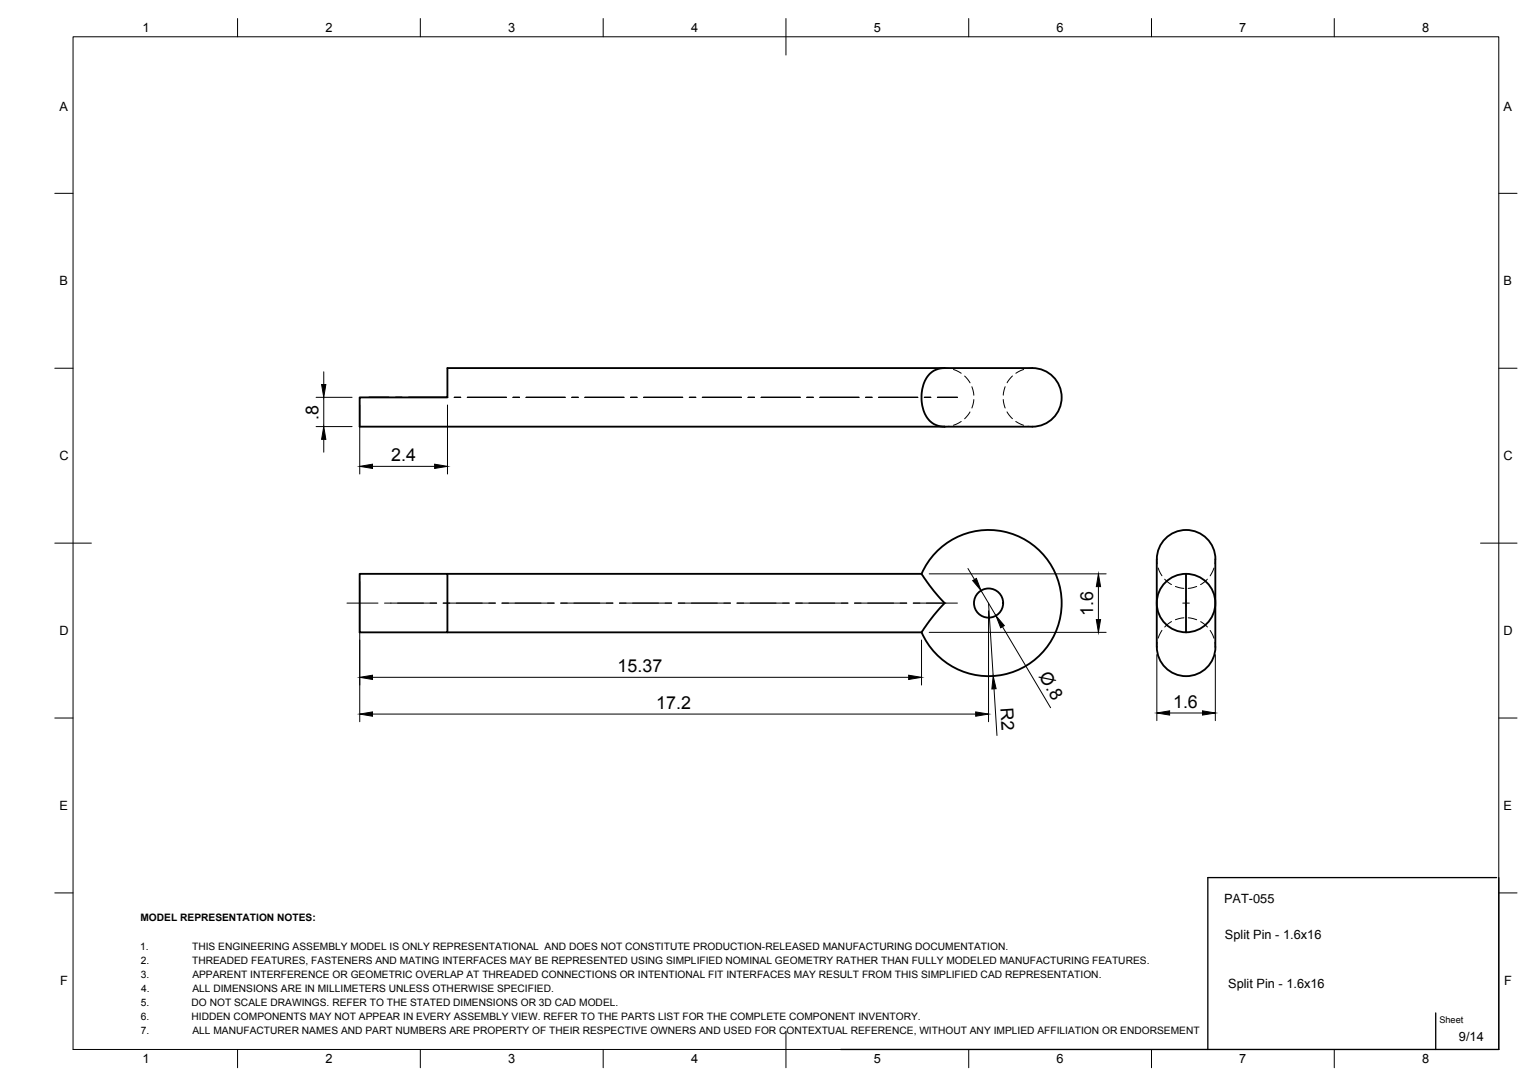
ISO-10303-21;
HEADER;
/* Generated by software containing ST-Developer
 * from STEP Tools, Inc. (www.steptools.com) 
 */

FILE_DESCRIPTION(
/* description */ ('Hinged panel with latch'),
/* implementation_level */ '2;1');

FILE_NAME(
/* name */ 'Split Pin - 1.6x16.step',
/* time_stamp */ '2026-10-27T20:36:01-07:00',
/* author */ (''),
/* organization */ (''),
/* preprocessor_version */ 'ST-DEVELOPER v20.2',
/* originating_system */ 'Autodesk Translation Framework v15.17.0.0',
/* authorisation */ '');

FILE_SCHEMA (('AUTOMOTIVE_DESIGN { 1 0 10303 214 3 1 1 }'));
ENDSEC;

DATA;
#10=MECHANICAL_DESIGN_GEOMETRIC_PRESENTATION_REPRESENTATION('',(#301),#6743);
#239=TOROIDAL_SURFACE('',#4113,0.12,0.08);
#262=B_SPLINE_CURVE_WITH_KNOTS('',3,(#5988,#5989,#5990,#5991,#5992,#5993,
#5994,#5995,#5996,#5997,#5998,#5999,#6000,#6001,#6002,#6003,#6004,#6005,
#6006,#6007,#6008,#6009,#6010,#6011,#6012,#6013),.UNSPECIFIED.,.F.,.F.,
(4,2,2,2,2,2,2,2,2,2,2,2,4),(-0.00054581412719389,0.,0.0281583564005144,
0.0618496465371181,0.0905865724114538,0.120694112793616,0.144966158459363,
0.16923820412511,0.199345744507272,0.228082670381608,0.261773960518212,
0.289932316918681,0.290478131045882),.UNSPECIFIED.);
#263=B_SPLINE_CURVE_WITH_KNOTS('',3,(#6014,#6015,#6016,#6017,#6018,#6019,
#6020,#6021,#6022,#6023,#6024,#6025,#6026,#6027,#6028,#6029,#6030,#6031,
#6032,#6033,#6034,#6035,#6036,#6037,#6038,#6039),.UNSPECIFIED.,.F.,.F.,
(4,2,2,2,2,2,2,2,2,2,2,2,4),(-0.000545814127196571,0.,0.0281583564006391,
0.0618496465374156,0.0905865724118984,0.120694112794215,0.144966158460086,
0.169238204125958,0.199345744508275,0.228082670382758,0.261773960519534,
0.289932316920171,0.29047813104737),.UNSPECIFIED.);
#269=SHAPE_REPRESENTATION_RELATIONSHIP('SRR','None',#6844,#285);
#285=ADVANCED_BREP_SHAPE_REPRESENTATION('',(#317),#6730);
#301=STYLED_ITEM('',(#7003),#317);
#317=MANIFOLD_SOLID_BREP('Body1',#3803);
#343=FACE_BOUND('',#831,.T.);
#439=PLANE('',#4116);
#440=PLANE('',#4118);
#441=PLANE('',#4122);
#606=FACE_OUTER_BOUND('',#830,.T.);
#607=FACE_OUTER_BOUND('',#832,.T.);
#608=FACE_OUTER_BOUND('',#833,.T.);
#609=FACE_OUTER_BOUND('',#834,.T.);
#610=FACE_OUTER_BOUND('',#835,.T.);
#830=EDGE_LOOP('',(#3024,#3025,#3026,#3027));
#831=EDGE_LOOP('',(#3028,#3029));
#832=EDGE_LOOP('',(#3030,#3031));
#833=EDGE_LOOP('',(#3032,#3033,#3034,#3035));
#834=EDGE_LOOP('',(#3036,#3037,#3038,#3039,#3040,#3041,#3042,#3043,#3044));
#835=EDGE_LOOP('',(#3045,#3046,#3047));
#1167=LINE('',#6044,#1525);
#1168=LINE('',#6047,#1526);
#1169=LINE('',#6049,#1527);
#1170=LINE('',#6050,#1528);
#1171=LINE('',#6054,#1529);
#1525=VECTOR('',#4797,1.);
#1526=VECTOR('',#4800,1.);
#1527=VECTOR('',#4801,1.);
#1528=VECTOR('',#4802,1.);
#1529=VECTOR('',#4807,0.08);
#1726=CIRCLE('',#4114,0.08);
#1727=CIRCLE('',#4115,0.04);
#1728=CIRCLE('',#4117,0.08);
#1729=CIRCLE('',#4120,0.08);
#1730=CIRCLE('',#4121,0.08);
#1935=VERTEX_POINT('',#5983);
#1936=VERTEX_POINT('',#5986);
#1937=VERTEX_POINT('',#5987);
#1938=VERTEX_POINT('',#6041);
#1939=VERTEX_POINT('',#6042);
#1940=VERTEX_POINT('',#6046);
#1941=VERTEX_POINT('',#6048);
#1942=VERTEX_POINT('',#6052);
#2324=EDGE_CURVE('',#1935,#1935,#1726,.T.);
#2325=EDGE_CURVE('',#1935,#1935,#1727,.T.);
#2326=EDGE_CURVE('',#1936,#1937,#262,.T.);
#2327=EDGE_CURVE('',#1937,#1936,#263,.T.);
#2328=EDGE_CURVE('',#1938,#1939,#1728,.T.);
#2329=EDGE_CURVE('',#1938,#1939,#1167,.T.);
#2330=EDGE_CURVE('',#1939,#1940,#1168,.T.);
#2331=EDGE_CURVE('',#1941,#1940,#1169,.T.);
#2332=EDGE_CURVE('',#1938,#1941,#1170,.T.);
#2333=EDGE_CURVE('',#1942,#1941,#1729,.T.);
#2334=EDGE_CURVE('',#1942,#1937,#1171,.T.);
#2335=EDGE_CURVE('',#1940,#1942,#1730,.T.);
#3024=ORIENTED_EDGE('',*,*,#2324,.F.);
#3025=ORIENTED_EDGE('',*,*,#2325,.T.);
#3026=ORIENTED_EDGE('',*,*,#2324,.T.);
#3027=ORIENTED_EDGE('',*,*,#2325,.F.);
#3028=ORIENTED_EDGE('',*,*,#2326,.F.);
#3029=ORIENTED_EDGE('',*,*,#2327,.F.);
#3030=ORIENTED_EDGE('',*,*,#2328,.T.);
#3031=ORIENTED_EDGE('',*,*,#2329,.F.);
#3032=ORIENTED_EDGE('',*,*,#2329,.T.);
#3033=ORIENTED_EDGE('',*,*,#2330,.T.);
#3034=ORIENTED_EDGE('',*,*,#2331,.F.);
#3035=ORIENTED_EDGE('',*,*,#2332,.F.);
#3036=ORIENTED_EDGE('',*,*,#2328,.F.);
#3037=ORIENTED_EDGE('',*,*,#2332,.T.);
#3038=ORIENTED_EDGE('',*,*,#2333,.F.);
#3039=ORIENTED_EDGE('',*,*,#2334,.T.);
#3040=ORIENTED_EDGE('',*,*,#2327,.T.);
#3041=ORIENTED_EDGE('',*,*,#2326,.T.);
#3042=ORIENTED_EDGE('',*,*,#2334,.F.);
#3043=ORIENTED_EDGE('',*,*,#2335,.F.);
#3044=ORIENTED_EDGE('',*,*,#2330,.F.);
#3045=ORIENTED_EDGE('',*,*,#2335,.T.);
#3046=ORIENTED_EDGE('',*,*,#2333,.T.);
#3047=ORIENTED_EDGE('',*,*,#2331,.T.);
#3570=CYLINDRICAL_SURFACE('',#4119,0.08);
#3675=ADVANCED_FACE('',(#606,#343),#239,.T.);
#3676=ADVANCED_FACE('',(#607),#439,.F.);
#3677=ADVANCED_FACE('',(#608),#440,.T.);
#3678=ADVANCED_FACE('',(#609),#3570,.T.);
#3679=ADVANCED_FACE('',(#610),#441,.F.);
#3803=CLOSED_SHELL('',(#3675,#3676,#3677,#3678,#3679));
#4112=AXIS2_PLACEMENT_3D('',#5981,#4785,#4786);
#4113=AXIS2_PLACEMENT_3D('',#5982,#4787,#4788);
#4114=AXIS2_PLACEMENT_3D('',#5984,#4789,#4790);
#4115=AXIS2_PLACEMENT_3D('',#5985,#4791,#4792);
#4116=AXIS2_PLACEMENT_3D('',#6040,#4793,#4794);
#4117=AXIS2_PLACEMENT_3D('',#6043,#4795,#4796);
#4118=AXIS2_PLACEMENT_3D('',#6045,#4798,#4799);
#4119=AXIS2_PLACEMENT_3D('',#6051,#4803,#4804);
#4120=AXIS2_PLACEMENT_3D('',#6053,#4805,#4806);
#4121=AXIS2_PLACEMENT_3D('',#6055,#4808,#4809);
#4122=AXIS2_PLACEMENT_3D('',#6056,#4810,#4811);
#4785=DIRECTION('axis',(0.,0.,1.));
#4786=DIRECTION('refdir',(1.,0.,0.));
#4787=DIRECTION('center_axis',(-1.,0.,0.));
#4788=DIRECTION('ref_axis',(0.,0.,1.));
#4789=DIRECTION('center_axis',(0.,-1.,1.38777878078145E-16));
#4790=DIRECTION('ref_axis',(0.,-1.38777878078145E-16,-1.));
#4791=DIRECTION('center_axis',(1.,0.,0.));
#4792=DIRECTION('ref_axis',(0.,0.,1.));
#4793=DIRECTION('center_axis',(0.,1.,0.));
#4794=DIRECTION('ref_axis',(1.,0.,0.));
#4795=DIRECTION('center_axis',(0.,-1.,0.));
#4796=DIRECTION('ref_axis',(1.,0.,0.));
#4797=DIRECTION('',(0.,0.,1.));
#4798=DIRECTION('center_axis',(1.,0.,0.));
#4799=DIRECTION('ref_axis',(0.,0.,1.));
#4800=DIRECTION('',(0.,-1.,0.));
#4801=DIRECTION('',(0.,0.,1.));
#4802=DIRECTION('',(0.,-1.,0.));
#4803=DIRECTION('center_axis',(0.,-1.,0.));
#4804=DIRECTION('ref_axis',(1.,0.,0.));
#4805=DIRECTION('center_axis',(0.,-1.,0.));
#4806=DIRECTION('ref_axis',(1.,0.,0.));
#4807=DIRECTION('',(0.,1.,0.));
#4808=DIRECTION('center_axis',(0.,-1.,0.));
#4809=DIRECTION('ref_axis',(1.,0.,0.));
#4810=DIRECTION('center_axis',(0.,1.,0.));
#4811=DIRECTION('ref_axis',(1.,0.,0.));
#5981=CARTESIAN_POINT('',(0.,0.,0.));
#5982=CARTESIAN_POINT('Origin',(0.,0.12,0.));
#5983=CARTESIAN_POINT('',(-9.79717439317883E-18,0.12,-0.04));
#5984=CARTESIAN_POINT('Origin',(0.,0.12,-0.12));
#5985=CARTESIAN_POINT('Origin',(9.79717439317883E-18,0.12,0.));
#5986=CARTESIAN_POINT('',(0.08,-4.89858719658941E-18,7.34788079488412E-18));
#5987=CARTESIAN_POINT('',(-0.08,-4.89858719658941E-18,7.34788079488412E-18));
#5988=CARTESIAN_POINT('Ctrl Pts',(0.08,-4.89858719658941E-18,7.34788079488412E-18));
#5989=CARTESIAN_POINT('Ctrl Pts',(0.08,-0.00012864962353541,0.000128649623535413));
#5990=CARTESIAN_POINT('Ctrl Pts',(0.0799996896739287,-0.00025719571182076,
0.000257402596003253));
#5991=CARTESIAN_POINT('Ctrl Pts',(0.0799669711262291,-0.00701193164572964,
0.00703384588894362));
#5992=CARTESIAN_POINT('Ctrl Pts',(0.0791054994909294,-0.0133457972655825,
0.0139383126556792));
#5993=CARTESIAN_POINT('Ctrl Pts',(0.0749700088488058,-0.0265076530862524,
0.0292212026164895));
#5994=CARTESIAN_POINT('Ctrl Pts',(0.0712702072865517,-0.0331317062461458,
0.0375603420117568));
#5995=CARTESIAN_POINT('Ctrl Pts',(0.0612858949407667,-0.0440683985740427,
0.0520545604187517));
#5996=CARTESIAN_POINT('Ctrl Pts',(0.0555090276731744,-0.0485199197794574,
0.0582717815295611));
#5997=CARTESIAN_POINT('Ctrl Pts',(0.0412398082144208,-0.0561090538733877,
0.0691638397919718));
#5998=CARTESIAN_POINT('Ctrl Pts',(0.0327878980890048,-0.059089642483296,
0.0736229049587921));
#5999=CARTESIAN_POINT('Ctrl Pts',(0.0159233027310102,-0.0625179833270725,
0.0787936360751706));
#6000=CARTESIAN_POINT('Ctrl Pts',(0.00801661414593076,-0.0633030277982336,
0.08));
#6001=CARTESIAN_POINT('Ctrl Pts',(-0.00801661414593074,-0.0633030277982336,
0.08));
#6002=CARTESIAN_POINT('Ctrl Pts',(-0.0159233027310102,-0.0625179833270726,
0.0787936360751706));
#6003=CARTESIAN_POINT('Ctrl Pts',(-0.0327878980890049,-0.059089642483296,
0.0736229049587921));
#6004=CARTESIAN_POINT('Ctrl Pts',(-0.0412398082144209,-0.0561090538733877,
0.0691638397919717));
#6005=CARTESIAN_POINT('Ctrl Pts',(-0.0555090276731744,-0.0485199197794574,
0.0582717815295611));
#6006=CARTESIAN_POINT('Ctrl Pts',(-0.0612858949407667,-0.0440683985740427,
0.0520545604187517));
#6007=CARTESIAN_POINT('Ctrl Pts',(-0.0712702072865517,-0.0331317062461458,
0.0375603420117568));
#6008=CARTESIAN_POINT('Ctrl Pts',(-0.0749700088488058,-0.0265076530862524,
0.0292212026164895));
#6009=CARTESIAN_POINT('Ctrl Pts',(-0.0791054994909264,-0.0133457972655921,
0.0139383126556903));
#6010=CARTESIAN_POINT('Ctrl Pts',(-0.0799669711262287,-0.00701193164579759,
0.0070338458890125));
#6011=CARTESIAN_POINT('Ctrl Pts',(-0.0799996896739287,-0.000257195711817665,
0.000257402596000083));
#6012=CARTESIAN_POINT('Ctrl Pts',(-0.08,-0.000128649623538514,0.000128649623538516));
#6013=CARTESIAN_POINT('Ctrl Pts',(-0.08,-4.89858719658941E-18,7.34788079488412E-18));
#6014=CARTESIAN_POINT('Ctrl Pts',(-0.08,-4.89858719658941E-18,7.34788079488412E-18));
#6015=CARTESIAN_POINT('Ctrl Pts',(-0.08,-0.000128649623536042,-0.00012864962353603));
#6016=CARTESIAN_POINT('Ctrl Pts',(-0.0799996896739287,-0.000257195711820127,
-0.000257402596002604));
#6017=CARTESIAN_POINT('Ctrl Pts',(-0.0799669711262289,-0.0070119316457589,
-0.00703384588897312));
#6018=CARTESIAN_POINT('Ctrl Pts',(-0.0791054994909281,-0.0133457972655867,
-0.0139383126556841));
#6019=CARTESIAN_POINT('Ctrl Pts',(-0.0749700088488058,-0.0265076530862525,
-0.0292212026164896));
#6020=CARTESIAN_POINT('Ctrl Pts',(-0.0712702072865516,-0.0331317062461459,
-0.0375603420117568));
#6021=CARTESIAN_POINT('Ctrl Pts',(-0.0612858949407667,-0.0440683985740427,
-0.0520545604187517));
#6022=CARTESIAN_POINT('Ctrl Pts',(-0.0555090276731744,-0.0485199197794574,
-0.0582717815295611));
#6023=CARTESIAN_POINT('Ctrl Pts',(-0.0412398082144209,-0.0561090538733877,
-0.0691638397919717));
#6024=CARTESIAN_POINT('Ctrl Pts',(-0.0327878980890049,-0.059089642483296,
-0.0736229049587921));
#6025=CARTESIAN_POINT('Ctrl Pts',(-0.0159233027310101,-0.0625179833270725,
-0.0787936360751706));
#6026=CARTESIAN_POINT('Ctrl Pts',(-0.00801661414593069,-0.0633030277982336,
-0.08));
#6027=CARTESIAN_POINT('Ctrl Pts',(0.0080166141459307,-0.0633030277982336,
-0.08));
#6028=CARTESIAN_POINT('Ctrl Pts',(0.0159233027310101,-0.0625179833270725,
-0.0787936360751706));
#6029=CARTESIAN_POINT('Ctrl Pts',(0.0327878980890049,-0.0590896424832959,
-0.0736229049587921));
#6030=CARTESIAN_POINT('Ctrl Pts',(0.0412398082144209,-0.0561090538733877,
-0.0691638397919717));
#6031=CARTESIAN_POINT('Ctrl Pts',(0.0555090276731744,-0.0485199197794574,
-0.0582717815295611));
#6032=CARTESIAN_POINT('Ctrl Pts',(0.0612858949407666,-0.0440683985740428,
-0.0520545604187518));
#6033=CARTESIAN_POINT('Ctrl Pts',(0.0712702072865517,-0.0331317062461458,
-0.0375603420117568));
#6034=CARTESIAN_POINT('Ctrl Pts',(0.0749700088488058,-0.0265076530862524,
-0.0292212026164895));
#6035=CARTESIAN_POINT('Ctrl Pts',(0.079105499490928,-0.013345797265587,
-0.0139383126556845));
#6036=CARTESIAN_POINT('Ctrl Pts',(0.0799669711262289,-0.00701193164576148,
-0.00703384588897579));
#6037=CARTESIAN_POINT('Ctrl Pts',(0.0799996896739287,-0.000257195711819584,
-0.000257402596002039));
#6038=CARTESIAN_POINT('Ctrl Pts',(0.08,-0.000128649623536605,-0.000128649623536593));
#6039=CARTESIAN_POINT('Ctrl Pts',(0.08,-4.89858719658941E-18,7.34788079488412E-18));
#6040=CARTESIAN_POINT('Origin',(0.04,-1.36,0.));
#6041=CARTESIAN_POINT('',(0.,-1.36,-0.08));
#6042=CARTESIAN_POINT('',(0.,-1.36,0.08));
#6043=CARTESIAN_POINT('Origin',(0.,-1.36,0.));
#6044=CARTESIAN_POINT('',(0.,-1.36,-0.04));
#6045=CARTESIAN_POINT('Origin',(0.,0.,-0.08));
#6046=CARTESIAN_POINT('',(0.,-1.6,0.08));
#6047=CARTESIAN_POINT('',(0.,0.,0.08));
#6048=CARTESIAN_POINT('',(0.,-1.6,-0.08));
#6049=CARTESIAN_POINT('',(0.,-1.6,-0.09));
#6050=CARTESIAN_POINT('',(0.,0.,-0.08));
#6051=CARTESIAN_POINT('Origin',(0.,0.,0.));
#6052=CARTESIAN_POINT('',(-0.08,-1.6,-9.79717439317883E-18));
#6053=CARTESIAN_POINT('Origin',(0.,-1.6,0.));
#6054=CARTESIAN_POINT('',(-0.08,0.,-9.79717439317883E-18));
#6055=CARTESIAN_POINT('Origin',(0.,-1.6,0.));
#6056=CARTESIAN_POINT('Origin',(-0.04,-1.6,0.));
#6709=UNCERTAINTY_MEASURE_WITH_UNIT(LENGTH_MEASURE(0.001),#6744,
'DISTANCE_ACCURACY_VALUE',
'Maximum model space distance between geometric entities at asserted c
onnectivities');
#6722=UNCERTAINTY_MEASURE_WITH_UNIT(LENGTH_MEASURE(0.001),#6744,
'DISTANCE_ACCURACY_VALUE',
'Maximum model space distance between geometric entities at asserted c
onnectivities');
#6730=(
GEOMETRIC_REPRESENTATION_CONTEXT(3)
GLOBAL_UNCERTAINTY_ASSIGNED_CONTEXT((#6709))
GLOBAL_UNIT_ASSIGNED_CONTEXT((#6744,#6746,#6747))
REPRESENTATION_CONTEXT('','3D')
);
#6743=(
GEOMETRIC_REPRESENTATION_CONTEXT(3)
GLOBAL_UNCERTAINTY_ASSIGNED_CONTEXT((#6722))
GLOBAL_UNIT_ASSIGNED_CONTEXT((#6744,#6746,#6747))
REPRESENTATION_CONTEXT('','3D')
);
#6744=(
LENGTH_UNIT()
NAMED_UNIT(*)
SI_UNIT(.CENTI.,.METRE.)
);
#6746=(
NAMED_UNIT(*)
PLANE_ANGLE_UNIT()
SI_UNIT($,.RADIAN.)
);
#6747=(
NAMED_UNIT(*)
SI_UNIT($,.STERADIAN.)
SOLID_ANGLE_UNIT()
);
#6755=SHAPE_DEFINITION_REPRESENTATION(#6775,#6844);
#6775=PRODUCT_DEFINITION_SHAPE('',$,#6865);
#6844=SHAPE_REPRESENTATION('',(#4112),#6730);
#6857=PRODUCT_DEFINITION_CONTEXT('part definition',#6919,'design');
#6865=PRODUCT_DEFINITION('Split Pin - 1.6x16','Split Pin - 1.6x16',#6885,
#6857);
#6885=PRODUCT_DEFINITION_FORMATION('',$,#6928);
#6919=APPLICATION_CONTEXT(
'Core Data for Automotive Mechanical Design Process');
#6920=PRODUCT_CONTEXT('part definition',#6919,'mechanical');
#6928=PRODUCT('Split Pin - 1.6x16','Split Pin - 1.6x16',
'Split Pin - 1.6x16',(#6920));
#6997=COLOUR_RGB('Grey',0.48,0.52,0.57);
#6998=FILL_AREA_STYLE_COLOUR('',#6997);
#6999=FILL_AREA_STYLE('',(#6998));
#7000=SURFACE_STYLE_FILL_AREA(#6999);
#7001=SURFACE_SIDE_STYLE('',(#7000));
#7002=SURFACE_STYLE_USAGE(.BOTH.,#7001);
#7003=PRESENTATION_STYLE_ASSIGNMENT((#7002));
ENDSEC;
END-ISO-10303-21;
